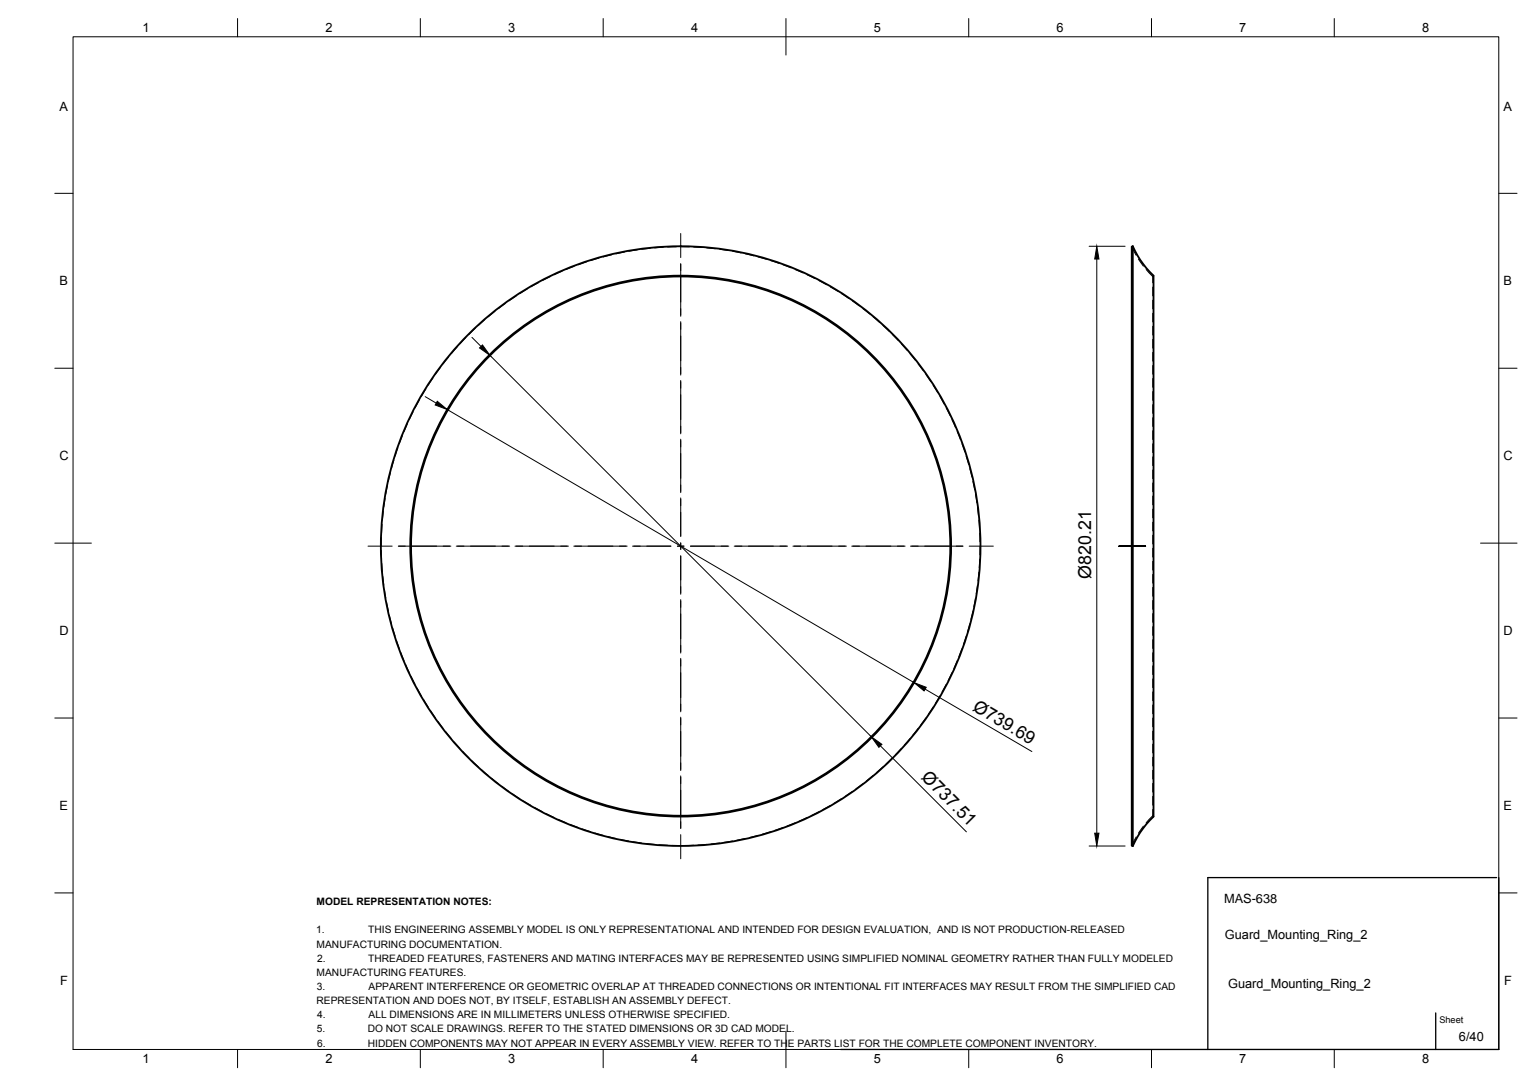
ISO-10303-21;
HEADER;
FILE_DESCRIPTION((''),'2;1');
FILE_NAME('Guard_Mounting_Ring_2.step','2026-10-09T12:00:21-07:00',(''),(''),'','','');
FILE_SCHEMA (('AUTOMOTIVE_DESIGN { 1 0 10303 214 3 1 1 }'));
ENDSEC;
DATA;
#10=MECHANICAL_DESIGN_GEOMETRIC_PRESENTATION_REPRESENTATION('',(#397),#10334);
#333=SHAPE_REPRESENTATION_RELATIONSHIP('SRR','None',#10449,#365) ;
#365=ADVANCED_BREP_SHAPE_REPRESENTATION('',(#437),#10301) ;
#397=STYLED_ITEM('',(#10631),#437) ;
#437=MANIFOLD_SOLID_BREP('Body1',#3559) ;
#533=LINE('',#5639,#691) ;
#534=LINE('',#5650,#692) ;
#691=VECTOR('',#4491,41.0104872556709) ;
#692=VECTOR('',#4506,36.984442871488) ;
#849=CONICAL_SURFACE('',#3965,41.0104872556709,0.416359756197082) ;
#850=CONICAL_SURFACE('',#3972,36.984442871488,0.81286797102658) ;
#855=FACE_OUTER_BOUND('',#1055,.T.) ;
#856=FACE_OUTER_BOUND('',#1056,.T.) ;
#857=FACE_OUTER_BOUND('',#1057,.T.) ;
#858=FACE_OUTER_BOUND('',#1058,.T.) ;
#1055=EDGE_LOOP('',(#2325,#2326,#2327,#2328,#2329,#2330)) ;
#1056=EDGE_LOOP('',(#2331,#2332,#2333,#2334,#2335,#2336)) ;
#1057=EDGE_LOOP('',(#2337,#2338,#2339,#2340,#2341,#2342)) ;
#1058=EDGE_LOOP('',(#2343,#2344,#2345,#2346,#2347,#2348)) ;
#1266=CIRCLE('',#3960,41.0104872556708) ;
#1267=CIRCLE('',#3961,41.0104872556708) ;
#1268=CIRCLE('',#3962,12.6169576826623) ;
#1269=CIRCLE('',#3963,36.984442871488) ;
#1270=CIRCLE('',#3964,36.984442871488) ;
#1271=CIRCLE('',#3966,40.9498221718178) ;
#1272=CIRCLE('',#3967,40.9498221718178) ;
#1273=CIRCLE('',#3969,36.8755027779276) ;
#1274=CIRCLE('',#3970,36.8755027779276) ;
#1275=CIRCLE('',#3971,12.7669576826623) ;
#1505=VERTEX_POINT('',#5628) ;
#1506=VERTEX_POINT('',#5629) ;
#1507=VERTEX_POINT('',#5632) ;
#1508=VERTEX_POINT('',#5634) ;
#1509=VERTEX_POINT('',#5638) ;
#1510=VERTEX_POINT('',#5640) ;
#1511=VERTEX_POINT('',#5644) ;
#1512=VERTEX_POINT('',#5645) ;
#1819=EDGE_CURVE('',#1505,#1506,#1266,.T.) ;
#1820=EDGE_CURVE('',#1506,#1505,#1267,.T.) ;
#1821=EDGE_CURVE('',#1506,#1507,#1268,.T.) ;
#1822=EDGE_CURVE('',#1507,#1508,#1269,.T.) ;
#1823=EDGE_CURVE('',#1508,#1507,#1270,.T.) ;
#1824=EDGE_CURVE('',#1505,#1509,#533,.T.) ;
#1825=EDGE_CURVE('',#1510,#1509,#1271,.T.) ;
#1826=EDGE_CURVE('',#1509,#1510,#1272,.T.) ;
#1827=EDGE_CURVE('',#1511,#1512,#1273,.T.) ;
#1828=EDGE_CURVE('',#1512,#1511,#1274,.T.) ;
#1829=EDGE_CURVE('',#1512,#1510,#1275,.T.) ;
#1830=EDGE_CURVE('',#1511,#1508,#534,.T.) ;
#2325=ORIENTED_EDGE('',*,*,#1819,.F.) ;
#2326=ORIENTED_EDGE('',*,*,#1820,.F.) ;
#2327=ORIENTED_EDGE('',*,*,#1821,.T.) ;
#2328=ORIENTED_EDGE('',*,*,#1822,.T.) ;
#2329=ORIENTED_EDGE('',*,*,#1823,.T.) ;
#2330=ORIENTED_EDGE('',*,*,#1821,.F.) ;
#2331=ORIENTED_EDGE('',*,*,#1819,.T.) ;
#2332=ORIENTED_EDGE('',*,*,#1820,.T.) ;
#2333=ORIENTED_EDGE('',*,*,#1824,.T.) ;
#2334=ORIENTED_EDGE('',*,*,#1825,.F.) ;
#2335=ORIENTED_EDGE('',*,*,#1826,.F.) ;
#2336=ORIENTED_EDGE('',*,*,#1824,.F.) ;
#2337=ORIENTED_EDGE('',*,*,#1827,.F.) ;
#2338=ORIENTED_EDGE('',*,*,#1828,.F.) ;
#2339=ORIENTED_EDGE('',*,*,#1829,.T.) ;
#2340=ORIENTED_EDGE('',*,*,#1825,.T.) ;
#2341=ORIENTED_EDGE('',*,*,#1826,.T.) ;
#2342=ORIENTED_EDGE('',*,*,#1829,.F.) ;
#2343=ORIENTED_EDGE('',*,*,#1827,.T.) ;
#2344=ORIENTED_EDGE('',*,*,#1828,.T.) ;
#2345=ORIENTED_EDGE('',*,*,#1830,.T.) ;
#2346=ORIENTED_EDGE('',*,*,#1822,.F.) ;
#2347=ORIENTED_EDGE('',*,*,#1823,.F.) ;
#2348=ORIENTED_EDGE('',*,*,#1830,.F.) ;
#3303=TOROIDAL_SURFACE('',#3959,46.1132125609321,12.6169576826623) ;
#3304=TOROIDAL_SURFACE('',#3968,46.1132125609321,12.7669576826623) ;
#3363=ADVANCED_FACE('',(#855),#3303,.F.) ;
#3364=ADVANCED_FACE('',(#856),#849,.T.) ;
#3365=ADVANCED_FACE('',(#857),#3304,.T.) ;
#3366=ADVANCED_FACE('',(#858),#850,.F.) ;
#3559=CLOSED_SHELL('',(#3363,#3364,#3365,#3366)) ;
#3958=AXIS2_PLACEMENT_3D('',#5626,#4475,#4476) ;
#3959=AXIS2_PLACEMENT_3D('',#5627,#4477,#4478) ;
#3960=AXIS2_PLACEMENT_3D('',#5630,#4479,#4480) ;
#3961=AXIS2_PLACEMENT_3D('',#5631,#4481,#4482) ;
#3962=AXIS2_PLACEMENT_3D('',#5633,#4483,#4484) ;
#3963=AXIS2_PLACEMENT_3D('',#5635,#4485,#4486) ;
#3964=AXIS2_PLACEMENT_3D('',#5636,#4487,#4488) ;
#3965=AXIS2_PLACEMENT_3D('',#5637,#4489,#4490) ;
#3966=AXIS2_PLACEMENT_3D('',#5641,#4492,#4493) ;
#3967=AXIS2_PLACEMENT_3D('',#5642,#4494,#4495) ;
#3968=AXIS2_PLACEMENT_3D('',#5643,#4496,#4497) ;
#3969=AXIS2_PLACEMENT_3D('',#5646,#4498,#4499) ;
#3970=AXIS2_PLACEMENT_3D('',#5647,#4500,#4501) ;
#3971=AXIS2_PLACEMENT_3D('',#5648,#4502,#4503) ;
#3972=AXIS2_PLACEMENT_3D('',#5649,#4504,#4505) ;
#4475=DIRECTION('axis',(0.,0.,1.)) ;
#4476=DIRECTION('refdir',(1.,0.,0.)) ;
#4477=DIRECTION('center_axis',(0.,-1.,0.)) ;
#4478=DIRECTION('ref_axis',(0.,0.,-1.)) ;
#4479=DIRECTION('center_axis',(0.,-1.,0.)) ;
#4480=DIRECTION('ref_axis',(0.,0.,-1.)) ;
#4481=DIRECTION('center_axis',(0.,-1.,0.)) ;
#4482=DIRECTION('ref_axis',(0.,0.,-1.)) ;
#4483=DIRECTION('center_axis',(1.,0.,1.20984279938742E-16)) ;
#4484=DIRECTION('ref_axis',(-1.20984279938742E-16,0.,1.)) ;
#4485=DIRECTION('center_axis',(0.,-1.,0.)) ;
#4486=DIRECTION('ref_axis',(0.,0.,-1.)) ;
#4487=DIRECTION('center_axis',(0.,-1.,0.)) ;
#4488=DIRECTION('ref_axis',(0.,0.,-1.)) ;
#4489=DIRECTION('center_axis',(0.,1.,0.)) ;
#4490=DIRECTION('ref_axis',(0.,0.,1.)) ;
#4491=DIRECTION('',(4.9528867173767E-17,-0.914567234661089,0.404433892353705)) ;
#4492=DIRECTION('center_axis',(0.,-1.,0.)) ;
#4493=DIRECTION('ref_axis',(0.,0.,-1.)) ;
#4494=DIRECTION('center_axis',(0.,-1.,0.)) ;
#4495=DIRECTION('ref_axis',(0.,0.,-1.)) ;
#4496=DIRECTION('center_axis',(0.,-1.,0.)) ;
#4497=DIRECTION('ref_axis',(0.,0.,-1.)) ;
#4498=DIRECTION('center_axis',(0.,-1.,0.)) ;
#4499=DIRECTION('ref_axis',(0.,0.,-1.)) ;
#4500=DIRECTION('center_axis',(0.,-1.,0.)) ;
#4501=DIRECTION('ref_axis',(0.,0.,-1.)) ;
#4502=DIRECTION('center_axis',(-1.,0.,-1.20676066801522E-16)) ;
#4503=DIRECTION('ref_axis',(-1.20676066801522E-16,0.,1.)) ;
#4504=DIRECTION('center_axis',(0.,1.,0.)) ;
#4505=DIRECTION('ref_axis',(0.,0.,1.)) ;
#4506=DIRECTION('',(-8.89414010484684E-17,0.687418365519119,-0.72626165446554)) ;
#5626=CARTESIAN_POINT('',(0.,0.,0.)) ;
#5627=CARTESIAN_POINT('Origin',(23.47768801576,52.6592998081416,68.2224337400009)) ;
#5628=CARTESIAN_POINT('',(23.47768801576,41.1202437104732,27.21194648433)) ;
#5629=CARTESIAN_POINT('',(23.47768801576,41.1202437104732,109.232920995672)) ;
#5630=CARTESIAN_POINT('Origin',(23.47768801576,41.1202437104732,68.2224337400009)) ;
#5631=CARTESIAN_POINT('Origin',(23.47768801576,41.1202437104732,68.2224337400009)) ;
#5632=CARTESIAN_POINT('',(23.47768801576,43.9499264022543,105.206876611489)) ;
#5633=CARTESIAN_POINT('Origin',(23.47768801576,52.6592998081416,114.335646300933)) ;
#5634=CARTESIAN_POINT('',(23.47768801576,43.9499264022543,31.2379908685129)) ;
#5635=CARTESIAN_POINT('Origin',(23.47768801576,43.9499264022543,68.2224337400009)) ;
#5636=CARTESIAN_POINT('Origin',(23.47768801576,43.9499264022543,68.2224337400009)) ;
#5637=CARTESIAN_POINT('Origin',(23.47768801576,41.1202437104732,68.2224337400009)) ;
#5638=CARTESIAN_POINT('',(23.47768801576,40.9830586252741,27.272611568183)) ;
#5639=CARTESIAN_POINT('',(23.47768801576,41.1202437104732,27.21194648433)) ;
#5640=CARTESIAN_POINT('',(23.47768801576,40.9830586252741,109.172255911819)) ;
#5641=CARTESIAN_POINT('Origin',(23.47768801576,40.9830586252741,68.2224337400009)) ;
#5642=CARTESIAN_POINT('Origin',(23.47768801576,40.9830586252741,68.2224337400009)) ;
#5643=CARTESIAN_POINT('Origin',(23.47768801576,52.6592998081416,68.2224337400009)) ;
#5644=CARTESIAN_POINT('',(23.47768801576,43.8468128472507,31.3469309620732)) ;
#5645=CARTESIAN_POINT('',(23.47768801576,43.8468128472507,105.097936517929)) ;
#5646=CARTESIAN_POINT('Origin',(23.47768801576,43.8468128472507,68.2224337400009)) ;
#5647=CARTESIAN_POINT('Origin',(23.47768801576,43.8468128472507,68.2224337400009)) ;
#5648=CARTESIAN_POINT('Origin',(23.47768801576,52.6592998081416,114.335646300933)) ;
#5649=CARTESIAN_POINT('Origin',(23.47768801576,43.9499264022543,68.2224337400009)) ;
#5650=CARTESIAN_POINT('',(23.47768801576,43.9499264022543,31.2379908685129)) ;
#10264=UNCERTAINTY_MEASURE_WITH_UNIT(LENGTH_MEASURE(0.001),#10335,
'DISTANCE_ACCURACY_VALUE',
'Maximum model space distance between geometric entities at asserted c
onnectivities') ;
#10297=UNCERTAINTY_MEASURE_WITH_UNIT(LENGTH_MEASURE(0.001),#10335,
'DISTANCE_ACCURACY_VALUE',
'Maximum model space distance between geometric entities at asserted c
onnectivities') ;
#10301=(
GEOMETRIC_REPRESENTATION_CONTEXT(3)
GLOBAL_UNCERTAINTY_ASSIGNED_CONTEXT((#10264))
GLOBAL_UNIT_ASSIGNED_CONTEXT((#10335,#10337,#10338))
REPRESENTATION_CONTEXT('','3D')
) ;
#10334=(
GEOMETRIC_REPRESENTATION_CONTEXT(3)
GLOBAL_UNCERTAINTY_ASSIGNED_CONTEXT((#10297))
GLOBAL_UNIT_ASSIGNED_CONTEXT((#10335,#10337,#10338))
REPRESENTATION_CONTEXT('','3D')
) ;
#10335=(
LENGTH_UNIT()
NAMED_UNIT(*)
SI_UNIT(.CENTI.,.METRE.)
) ;
#10337=(
NAMED_UNIT(*)
PLANE_ANGLE_UNIT()
SI_UNIT($,.RADIAN.)
) ;
#10338=(
NAMED_UNIT(*)
SI_UNIT($,.STERADIAN.)
SOLID_ANGLE_UNIT()
) ;
#10342=SHAPE_DEFINITION_REPRESENTATION(#10378,#10449) ;
#10378=PRODUCT_DEFINITION_SHAPE('',$,#10486) ;
#10449=SHAPE_REPRESENTATION('',(#3958),#10301) ;
#10482=PRODUCT_DEFINITION_CONTEXT('part definition',#10592,'design') ;
#10486=PRODUCT_DEFINITION('Guard_Mounting_Ring_2',
'Guard_Mounting_Ring_2',#10522,#10482) ;
#10522=PRODUCT_DEFINITION_FORMATION('',$,#10597) ;
#10592=APPLICATION_CONTEXT(
'Core Data for Automotive Mechanical Design Process') ;
#10593=PRODUCT_CONTEXT('part definition',#10592,'mechanical') ;
#10597=PRODUCT('Guard_Mounting_Ring_2','Guard_Mounting_Ring_2',$,(#10593)) ;
#10631=PRESENTATION_STYLE_ASSIGNMENT((#10635)) ;
#10635=SURFACE_STYLE_USAGE(.BOTH.,#10639) ;
#10639=SURFACE_SIDE_STYLE('',(#10643)) ;
#10643=SURFACE_STYLE_FILL_AREA(#10647) ;
#10647=FILL_AREA_STYLE('Opaque(25,25,25)',(#10651)) ;
#10651=FILL_AREA_STYLE_COLOUR('Opaque(25,25,25)',#10655) ;
#10655=COLOUR_RGB('Opaque(25,25,25)', 0.09019608, 0.27058824, 0.51372549) ;
ENDSEC;
END-ISO-10303-21;
